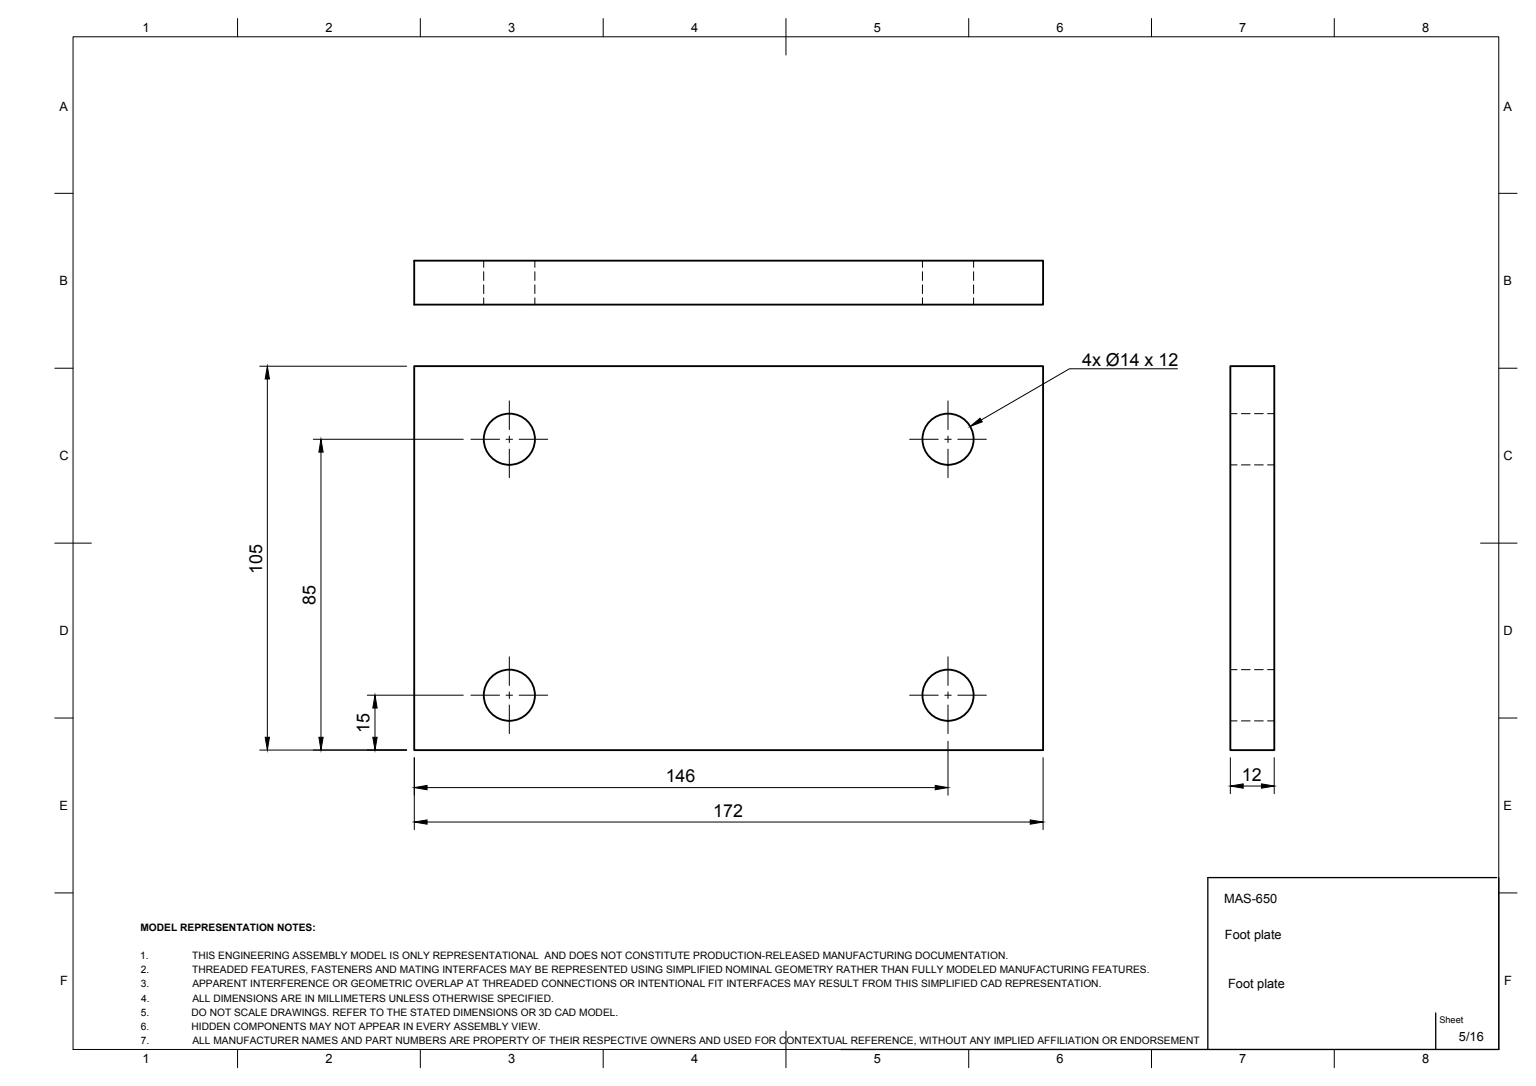
ISO-10303-21;
HEADER;
/* Generated by software containing ST-Developer
 * from STEP Tools, Inc. (www.steptools.com) 
 */

FILE_DESCRIPTION(
/* description */ ('Independent manual traversing gantry with native reusable aluminum pr
ofiles,180mm captured carriage travel, four bronze-bushed rollers, lin
ked ideal rolling motion, bonded acetal lateral guides, positive welde
d end stops and fully retained axle stacks. Editable native profile cu
t lengths220/400mm. Tool attachments viaM6 bridge-plate taps; mounted 
tool outside assembly. Welds, anchors, adhesives, fits, traction, load
/speed/structural/life ratings unassigned.'),
/* implementation_level */ '2;1');

FILE_NAME(
/* name */ 'Foot plate.step',
/* time_stamp */ '2026-11-09T20:04:38-08:00',
/* author */ (''),
/* organization */ (''),
/* preprocessor_version */ 'ST-DEVELOPER v20.2',
/* originating_system */ 'Autodesk Translation Framework v15.17.0.0',
/* authorisation */ '');

FILE_SCHEMA (('AUTOMOTIVE_DESIGN { 1 0 10303 214 3 1 1 }'));
ENDSEC;

DATA;
#10=MECHANICAL_DESIGN_GEOMETRIC_PRESENTATION_REPRESENTATION('',(#473),#13231);
#441=SHAPE_REPRESENTATION_RELATIONSHIP('SRR','None',#13330,#457);
#457=ADVANCED_BREP_SHAPE_REPRESENTATION('',(#489),#13217);
#473=STYLED_ITEM('',(#13419),#489);
#489=MANIFOLD_SOLID_BREP('Body1',#4153);
#507=FACE_BOUND('',#903,.T.);
#508=FACE_BOUND('',#904,.T.);
#509=FACE_BOUND('',#905,.T.);
#510=FACE_BOUND('',#906,.T.);
#511=FACE_BOUND('',#908,.T.);
#512=FACE_BOUND('',#909,.T.);
#513=FACE_BOUND('',#910,.T.);
#514=FACE_BOUND('',#911,.T.);
#572=PLANE('',#4428);
#573=PLANE('',#4429);
#574=PLANE('',#4430);
#575=PLANE('',#4431);
#576=PLANE('',#4432);
#577=PLANE('',#4433);
#669=FACE_OUTER_BOUND('',#894,.T.);
#670=FACE_OUTER_BOUND('',#895,.T.);
#671=FACE_OUTER_BOUND('',#896,.T.);
#672=FACE_OUTER_BOUND('',#897,.T.);
#673=FACE_OUTER_BOUND('',#898,.T.);
#674=FACE_OUTER_BOUND('',#899,.T.);
#675=FACE_OUTER_BOUND('',#900,.T.);
#676=FACE_OUTER_BOUND('',#901,.T.);
#677=FACE_OUTER_BOUND('',#902,.T.);
#678=FACE_OUTER_BOUND('',#907,.T.);
#894=EDGE_LOOP('',(#2874,#2875,#2876,#2877));
#895=EDGE_LOOP('',(#2878,#2879,#2880,#2881));
#896=EDGE_LOOP('',(#2882,#2883,#2884,#2885));
#897=EDGE_LOOP('',(#2886,#2887,#2888,#2889));
#898=EDGE_LOOP('',(#2890,#2891,#2892,#2893));
#899=EDGE_LOOP('',(#2894,#2895,#2896,#2897));
#900=EDGE_LOOP('',(#2898,#2899,#2900,#2901));
#901=EDGE_LOOP('',(#2902,#2903,#2904,#2905));
#902=EDGE_LOOP('',(#2906,#2907,#2908,#2909));
#903=EDGE_LOOP('',(#2910));
#904=EDGE_LOOP('',(#2911));
#905=EDGE_LOOP('',(#2912));
#906=EDGE_LOOP('',(#2913));
#907=EDGE_LOOP('',(#2914,#2915,#2916,#2917));
#908=EDGE_LOOP('',(#2918));
#909=EDGE_LOOP('',(#2919));
#910=EDGE_LOOP('',(#2920));
#911=EDGE_LOOP('',(#2921));
#1188=LINE('',#5983,#1450);
#1189=LINE('',#5989,#1451);
#1190=LINE('',#5995,#1452);
#1191=LINE('',#6001,#1453);
#1192=LINE('',#6006,#1454);
#1193=LINE('',#6008,#1455);
#1194=LINE('',#6010,#1456);
#1195=LINE('',#6011,#1457);
#1196=LINE('',#6014,#1458);
#1197=LINE('',#6016,#1459);
#1198=LINE('',#6017,#1460);
#1199=LINE('',#6020,#1461);
#1200=LINE('',#6022,#1462);
#1201=LINE('',#6023,#1463);
#1202=LINE('',#6025,#1464);
#1203=LINE('',#6026,#1465);
#1450=VECTOR('',#4947,7.);
#1451=VECTOR('',#4954,7.);
#1452=VECTOR('',#4961,7.);
#1453=VECTOR('',#4968,7.);
#1454=VECTOR('',#4973,10.);
#1455=VECTOR('',#4974,10.);
#1456=VECTOR('',#4975,10.);
#1457=VECTOR('',#4976,10.);
#1458=VECTOR('',#4979,10.);
#1459=VECTOR('',#4980,10.);
#1460=VECTOR('',#4981,10.);
#1461=VECTOR('',#4984,10.);
#1462=VECTOR('',#4985,10.);
#1463=VECTOR('',#4986,10.);
#1464=VECTOR('',#4989,10.);
#1465=VECTOR('',#4990,10.);
#1680=CIRCLE('',#4417,7.);
#1681=CIRCLE('',#4418,7.);
#1682=CIRCLE('',#4420,7.);
#1683=CIRCLE('',#4421,7.);
#1684=CIRCLE('',#4423,7.);
#1685=CIRCLE('',#4424,7.);
#1686=CIRCLE('',#4426,7.);
#1687=CIRCLE('',#4427,7.);
#1816=VERTEX_POINT('',#5980);
#1817=VERTEX_POINT('',#5982);
#1818=VERTEX_POINT('',#5986);
#1819=VERTEX_POINT('',#5988);
#1820=VERTEX_POINT('',#5992);
#1821=VERTEX_POINT('',#5994);
#1822=VERTEX_POINT('',#5998);
#1823=VERTEX_POINT('',#6000);
#1824=VERTEX_POINT('',#6004);
#1825=VERTEX_POINT('',#6005);
#1826=VERTEX_POINT('',#6007);
#1827=VERTEX_POINT('',#6009);
#1828=VERTEX_POINT('',#6013);
#1829=VERTEX_POINT('',#6015);
#1830=VERTEX_POINT('',#6019);
#1831=VERTEX_POINT('',#6021);
#2220=EDGE_CURVE('',#1816,#1816,#1680,.T.);
#2221=EDGE_CURVE('',#1816,#1817,#1188,.T.);
#2222=EDGE_CURVE('',#1817,#1817,#1681,.T.);
#2223=EDGE_CURVE('',#1818,#1818,#1682,.T.);
#2224=EDGE_CURVE('',#1818,#1819,#1189,.T.);
#2225=EDGE_CURVE('',#1819,#1819,#1683,.T.);
#2226=EDGE_CURVE('',#1820,#1820,#1684,.T.);
#2227=EDGE_CURVE('',#1820,#1821,#1190,.T.);
#2228=EDGE_CURVE('',#1821,#1821,#1685,.T.);
#2229=EDGE_CURVE('',#1822,#1822,#1686,.T.);
#2230=EDGE_CURVE('',#1822,#1823,#1191,.T.);
#2231=EDGE_CURVE('',#1823,#1823,#1687,.T.);
#2232=EDGE_CURVE('',#1824,#1825,#1192,.F.);
#2233=EDGE_CURVE('',#1825,#1826,#1193,.T.);
#2234=EDGE_CURVE('',#1827,#1826,#1194,.F.);
#2235=EDGE_CURVE('',#1824,#1827,#1195,.F.);
#2236=EDGE_CURVE('',#1828,#1824,#1196,.F.);
#2237=EDGE_CURVE('',#1829,#1827,#1197,.F.);
#2238=EDGE_CURVE('',#1828,#1829,#1198,.T.);
#2239=EDGE_CURVE('',#1830,#1828,#1199,.F.);
#2240=EDGE_CURVE('',#1831,#1829,#1200,.F.);
#2241=EDGE_CURVE('',#1830,#1831,#1201,.F.);
#2242=EDGE_CURVE('',#1825,#1830,#1202,.T.);
#2243=EDGE_CURVE('',#1826,#1831,#1203,.T.);
#2874=ORIENTED_EDGE('',*,*,#2220,.F.);
#2875=ORIENTED_EDGE('',*,*,#2221,.T.);
#2876=ORIENTED_EDGE('',*,*,#2222,.F.);
#2877=ORIENTED_EDGE('',*,*,#2221,.F.);
#2878=ORIENTED_EDGE('',*,*,#2223,.F.);
#2879=ORIENTED_EDGE('',*,*,#2224,.T.);
#2880=ORIENTED_EDGE('',*,*,#2225,.F.);
#2881=ORIENTED_EDGE('',*,*,#2224,.F.);
#2882=ORIENTED_EDGE('',*,*,#2226,.F.);
#2883=ORIENTED_EDGE('',*,*,#2227,.T.);
#2884=ORIENTED_EDGE('',*,*,#2228,.F.);
#2885=ORIENTED_EDGE('',*,*,#2227,.F.);
#2886=ORIENTED_EDGE('',*,*,#2229,.F.);
#2887=ORIENTED_EDGE('',*,*,#2230,.T.);
#2888=ORIENTED_EDGE('',*,*,#2231,.F.);
#2889=ORIENTED_EDGE('',*,*,#2230,.F.);
#2890=ORIENTED_EDGE('',*,*,#2232,.T.);
#2891=ORIENTED_EDGE('',*,*,#2233,.T.);
#2892=ORIENTED_EDGE('',*,*,#2234,.F.);
#2893=ORIENTED_EDGE('',*,*,#2235,.F.);
#2894=ORIENTED_EDGE('',*,*,#2236,.T.);
#2895=ORIENTED_EDGE('',*,*,#2235,.T.);
#2896=ORIENTED_EDGE('',*,*,#2237,.F.);
#2897=ORIENTED_EDGE('',*,*,#2238,.F.);
#2898=ORIENTED_EDGE('',*,*,#2239,.T.);
#2899=ORIENTED_EDGE('',*,*,#2238,.T.);
#2900=ORIENTED_EDGE('',*,*,#2240,.F.);
#2901=ORIENTED_EDGE('',*,*,#2241,.F.);
#2902=ORIENTED_EDGE('',*,*,#2242,.T.);
#2903=ORIENTED_EDGE('',*,*,#2241,.T.);
#2904=ORIENTED_EDGE('',*,*,#2243,.F.);
#2905=ORIENTED_EDGE('',*,*,#2233,.F.);
#2906=ORIENTED_EDGE('',*,*,#2243,.T.);
#2907=ORIENTED_EDGE('',*,*,#2240,.T.);
#2908=ORIENTED_EDGE('',*,*,#2237,.T.);
#2909=ORIENTED_EDGE('',*,*,#2234,.T.);
#2910=ORIENTED_EDGE('',*,*,#2220,.T.);
#2911=ORIENTED_EDGE('',*,*,#2223,.T.);
#2912=ORIENTED_EDGE('',*,*,#2226,.T.);
#2913=ORIENTED_EDGE('',*,*,#2229,.T.);
#2914=ORIENTED_EDGE('',*,*,#2242,.F.);
#2915=ORIENTED_EDGE('',*,*,#2232,.F.);
#2916=ORIENTED_EDGE('',*,*,#2236,.F.);
#2917=ORIENTED_EDGE('',*,*,#2239,.F.);
#2918=ORIENTED_EDGE('',*,*,#2222,.T.);
#2919=ORIENTED_EDGE('',*,*,#2225,.T.);
#2920=ORIENTED_EDGE('',*,*,#2228,.T.);
#2921=ORIENTED_EDGE('',*,*,#2231,.T.);
#3814=CYLINDRICAL_SURFACE('',#4416,7.);
#3815=CYLINDRICAL_SURFACE('',#4419,7.);
#3816=CYLINDRICAL_SURFACE('',#4422,7.);
#3817=CYLINDRICAL_SURFACE('',#4425,7.);
#3966=ADVANCED_FACE('',(#669),#3814,.F.);
#3967=ADVANCED_FACE('',(#670),#3815,.F.);
#3968=ADVANCED_FACE('',(#671),#3816,.F.);
#3969=ADVANCED_FACE('',(#672),#3817,.F.);
#3970=ADVANCED_FACE('',(#673),#572,.T.);
#3971=ADVANCED_FACE('',(#674),#573,.T.);
#3972=ADVANCED_FACE('',(#675),#574,.T.);
#3973=ADVANCED_FACE('',(#676),#575,.T.);
#3974=ADVANCED_FACE('',(#677,#507,#508,#509,#510),#576,.T.);
#3975=ADVANCED_FACE('',(#678,#511,#512,#513,#514),#577,.F.);
#4153=CLOSED_SHELL('',(#3966,#3967,#3968,#3969,#3970,#3971,#3972,#3973,
#3974,#3975));
#4415=AXIS2_PLACEMENT_3D('',#5978,#4941,#4942);
#4416=AXIS2_PLACEMENT_3D('',#5979,#4943,#4944);
#4417=AXIS2_PLACEMENT_3D('',#5981,#4945,#4946);
#4418=AXIS2_PLACEMENT_3D('',#5984,#4948,#4949);
#4419=AXIS2_PLACEMENT_3D('',#5985,#4950,#4951);
#4420=AXIS2_PLACEMENT_3D('',#5987,#4952,#4953);
#4421=AXIS2_PLACEMENT_3D('',#5990,#4955,#4956);
#4422=AXIS2_PLACEMENT_3D('',#5991,#4957,#4958);
#4423=AXIS2_PLACEMENT_3D('',#5993,#4959,#4960);
#4424=AXIS2_PLACEMENT_3D('',#5996,#4962,#4963);
#4425=AXIS2_PLACEMENT_3D('',#5997,#4964,#4965);
#4426=AXIS2_PLACEMENT_3D('',#5999,#4966,#4967);
#4427=AXIS2_PLACEMENT_3D('',#6002,#4969,#4970);
#4428=AXIS2_PLACEMENT_3D('',#6003,#4971,#4972);
#4429=AXIS2_PLACEMENT_3D('',#6012,#4977,#4978);
#4430=AXIS2_PLACEMENT_3D('',#6018,#4982,#4983);
#4431=AXIS2_PLACEMENT_3D('',#6024,#4987,#4988);
#4432=AXIS2_PLACEMENT_3D('',#6027,#4991,#4992);
#4433=AXIS2_PLACEMENT_3D('',#6028,#4993,#4994);
#4941=DIRECTION('axis',(0.,0.,1.));
#4942=DIRECTION('refdir',(1.,0.,0.));
#4943=DIRECTION('center_axis',(0.,0.,-1.));
#4944=DIRECTION('ref_axis',(1.,0.,0.));
#4945=DIRECTION('center_axis',(0.,0.,-1.));
#4946=DIRECTION('ref_axis',(1.,0.,0.));
#4947=DIRECTION('',(0.,0.,-1.));
#4948=DIRECTION('center_axis',(0.,0.,1.));
#4949=DIRECTION('ref_axis',(1.,0.,0.));
#4950=DIRECTION('center_axis',(0.,0.,-1.));
#4951=DIRECTION('ref_axis',(1.,0.,0.));
#4952=DIRECTION('center_axis',(0.,0.,-1.));
#4953=DIRECTION('ref_axis',(1.,0.,0.));
#4954=DIRECTION('',(0.,0.,-1.));
#4955=DIRECTION('center_axis',(0.,0.,1.));
#4956=DIRECTION('ref_axis',(1.,0.,0.));
#4957=DIRECTION('center_axis',(0.,0.,-1.));
#4958=DIRECTION('ref_axis',(1.,0.,0.));
#4959=DIRECTION('center_axis',(0.,0.,-1.));
#4960=DIRECTION('ref_axis',(1.,0.,0.));
#4961=DIRECTION('',(0.,0.,-1.));
#4962=DIRECTION('center_axis',(0.,0.,1.));
#4963=DIRECTION('ref_axis',(1.,0.,0.));
#4964=DIRECTION('center_axis',(0.,0.,-1.));
#4965=DIRECTION('ref_axis',(1.,0.,0.));
#4966=DIRECTION('center_axis',(0.,0.,-1.));
#4967=DIRECTION('ref_axis',(1.,0.,0.));
#4968=DIRECTION('',(0.,0.,-1.));
#4969=DIRECTION('center_axis',(0.,0.,1.));
#4970=DIRECTION('ref_axis',(1.,0.,0.));
#4971=DIRECTION('center_axis',(0.,1.,0.));
#4972=DIRECTION('ref_axis',(-1.,0.,0.));
#4973=DIRECTION('',(1.,0.,0.));
#4974=DIRECTION('',(0.,0.,1.));
#4975=DIRECTION('',(1.,0.,0.));
#4976=DIRECTION('',(0.,0.,-1.));
#4977=DIRECTION('center_axis',(1.,0.,0.));
#4978=DIRECTION('ref_axis',(0.,1.,0.));
#4979=DIRECTION('',(0.,-1.,0.));
#4980=DIRECTION('',(0.,-1.,0.));
#4981=DIRECTION('',(0.,0.,1.));
#4982=DIRECTION('center_axis',(0.,-1.,0.));
#4983=DIRECTION('ref_axis',(1.,0.,0.));
#4984=DIRECTION('',(-1.,0.,0.));
#4985=DIRECTION('',(-1.,0.,0.));
#4986=DIRECTION('',(0.,0.,-1.));
#4987=DIRECTION('center_axis',(-1.,0.,0.));
#4988=DIRECTION('ref_axis',(0.,-1.,0.));
#4989=DIRECTION('',(0.,-1.,0.));
#4990=DIRECTION('',(0.,-1.,0.));
#4991=DIRECTION('center_axis',(0.,0.,1.));
#4992=DIRECTION('ref_axis',(1.,0.,0.));
#4993=DIRECTION('center_axis',(0.,0.,1.));
#4994=DIRECTION('ref_axis',(1.,0.,0.));
#5978=CARTESIAN_POINT('',(0.,0.,0.));
#5979=CARTESIAN_POINT('Origin',(35.,-60.,6.));
#5980=CARTESIAN_POINT('',(28.,-60.,12.));
#5981=CARTESIAN_POINT('Origin',(35.,-60.,12.));
#5982=CARTESIAN_POINT('',(28.,-60.,0.));
#5983=CARTESIAN_POINT('',(28.,-60.,6.));
#5984=CARTESIAN_POINT('Origin',(35.,-60.,0.));
#5985=CARTESIAN_POINT('Origin',(-35.,-60.,6.));
#5986=CARTESIAN_POINT('',(-42.,-60.,12.));
#5987=CARTESIAN_POINT('Origin',(-35.,-60.,12.));
#5988=CARTESIAN_POINT('',(-42.,-60.,0.));
#5989=CARTESIAN_POINT('',(-42.,-60.,6.));
#5990=CARTESIAN_POINT('Origin',(-35.,-60.,0.));
#5991=CARTESIAN_POINT('Origin',(-35.,60.,6.));
#5992=CARTESIAN_POINT('',(-42.,60.,12.));
#5993=CARTESIAN_POINT('Origin',(-35.,60.,12.));
#5994=CARTESIAN_POINT('',(-42.,60.,0.));
#5995=CARTESIAN_POINT('',(-42.,60.,6.));
#5996=CARTESIAN_POINT('Origin',(-35.,60.,0.));
#5997=CARTESIAN_POINT('Origin',(35.,60.,6.));
#5998=CARTESIAN_POINT('',(28.,60.,12.));
#5999=CARTESIAN_POINT('Origin',(35.,60.,12.));
#6000=CARTESIAN_POINT('',(28.,60.,0.));
#6001=CARTESIAN_POINT('',(28.,60.,6.));
#6002=CARTESIAN_POINT('Origin',(35.,60.,0.));
#6003=CARTESIAN_POINT('Origin',(50.,86.,0.));
#6004=CARTESIAN_POINT('',(55.,86.,0.));
#6005=CARTESIAN_POINT('',(-50.,86.,0.));
#6006=CARTESIAN_POINT('',(25.,86.,0.));
#6007=CARTESIAN_POINT('',(-50.,86.,12.));
#6008=CARTESIAN_POINT('',(-50.,86.,0.));
#6009=CARTESIAN_POINT('',(55.,86.,12.));
#6010=CARTESIAN_POINT('',(25.,86.,12.));
#6011=CARTESIAN_POINT('',(55.,86.,0.));
#6012=CARTESIAN_POINT('Origin',(55.,-80.,0.));
#6013=CARTESIAN_POINT('',(55.,-86.,0.));
#6014=CARTESIAN_POINT('',(55.,-40.,0.));
#6015=CARTESIAN_POINT('',(55.,-86.,12.));
#6016=CARTESIAN_POINT('',(55.,-40.,12.));
#6017=CARTESIAN_POINT('',(55.,-86.,0.));
#6018=CARTESIAN_POINT('Origin',(-50.,-86.,0.));
#6019=CARTESIAN_POINT('',(-50.,-86.,0.));
#6020=CARTESIAN_POINT('',(-25.,-86.,0.));
#6021=CARTESIAN_POINT('',(-50.,-86.,12.));
#6022=CARTESIAN_POINT('',(-25.,-86.,12.));
#6023=CARTESIAN_POINT('',(-50.,-86.,0.));
#6024=CARTESIAN_POINT('Origin',(-50.,80.,0.));
#6025=CARTESIAN_POINT('',(-50.,80.,0.));
#6026=CARTESIAN_POINT('',(-50.,80.,12.));
#6027=CARTESIAN_POINT('Origin',(0.,0.,12.));
#6028=CARTESIAN_POINT('Origin',(0.,0.,0.));
#13199=UNCERTAINTY_MEASURE_WITH_UNIT(LENGTH_MEASURE(0.01),#13232,
'DISTANCE_ACCURACY_VALUE',
'Maximum model space distance between geometric entities at asserted c
onnectivities');
#13213=UNCERTAINTY_MEASURE_WITH_UNIT(LENGTH_MEASURE(0.01),#13232,
'DISTANCE_ACCURACY_VALUE',
'Maximum model space distance between geometric entities at asserted c
onnectivities');
#13217=(
GEOMETRIC_REPRESENTATION_CONTEXT(3)
GLOBAL_UNCERTAINTY_ASSIGNED_CONTEXT((#13199))
GLOBAL_UNIT_ASSIGNED_CONTEXT((#13232,#13234,#13235))
REPRESENTATION_CONTEXT('','3D')
);
#13231=(
GEOMETRIC_REPRESENTATION_CONTEXT(3)
GLOBAL_UNCERTAINTY_ASSIGNED_CONTEXT((#13213))
GLOBAL_UNIT_ASSIGNED_CONTEXT((#13232,#13234,#13235))
REPRESENTATION_CONTEXT('','3D')
);
#13232=(
LENGTH_UNIT()
NAMED_UNIT(*)
SI_UNIT(.MILLI.,.METRE.)
);
#13234=(
NAMED_UNIT(*)
PLANE_ANGLE_UNIT()
SI_UNIT($,.RADIAN.)
);
#13235=(
NAMED_UNIT(*)
SI_UNIT($,.STERADIAN.)
SOLID_ANGLE_UNIT()
);
#13239=SHAPE_DEFINITION_REPRESENTATION(#13256,#13330);
#13256=PRODUCT_DEFINITION_SHAPE('',$,#13348);
#13330=SHAPE_REPRESENTATION('',(#4415),#13217);
#13344=PRODUCT_DEFINITION_CONTEXT('part definition',#13397,'design');
#13348=PRODUCT_DEFINITION('Foot plate','Foot plate',#13365,#13344);
#13365=PRODUCT_DEFINITION_FORMATION('',$,#13402);
#13397=APPLICATION_CONTEXT(
'Core Data for Automotive Mechanical Design Process');
#13398=PRODUCT_CONTEXT('part definition',#13397,'mechanical');
#13402=PRODUCT('Foot plate','Foot plate',$,(#13398));
#13419=PRESENTATION_STYLE_ASSIGNMENT((#13433));
#13433=SURFACE_STYLE_USAGE(.BOTH.,#13447);
#13447=SURFACE_SIDE_STYLE('',(#13461));
#13461=SURFACE_STYLE_FILL_AREA(#13475);
#13475=FILL_AREA_STYLE('Foot gray',(#13489));
#13489=FILL_AREA_STYLE_COLOUR('Foot gray',#13503);
#13503=COLOUR_RGB('Foot gray',0.576470588235294,0.615686274509804,0.666666666666667);
ENDSEC;
END-ISO-10303-21;
